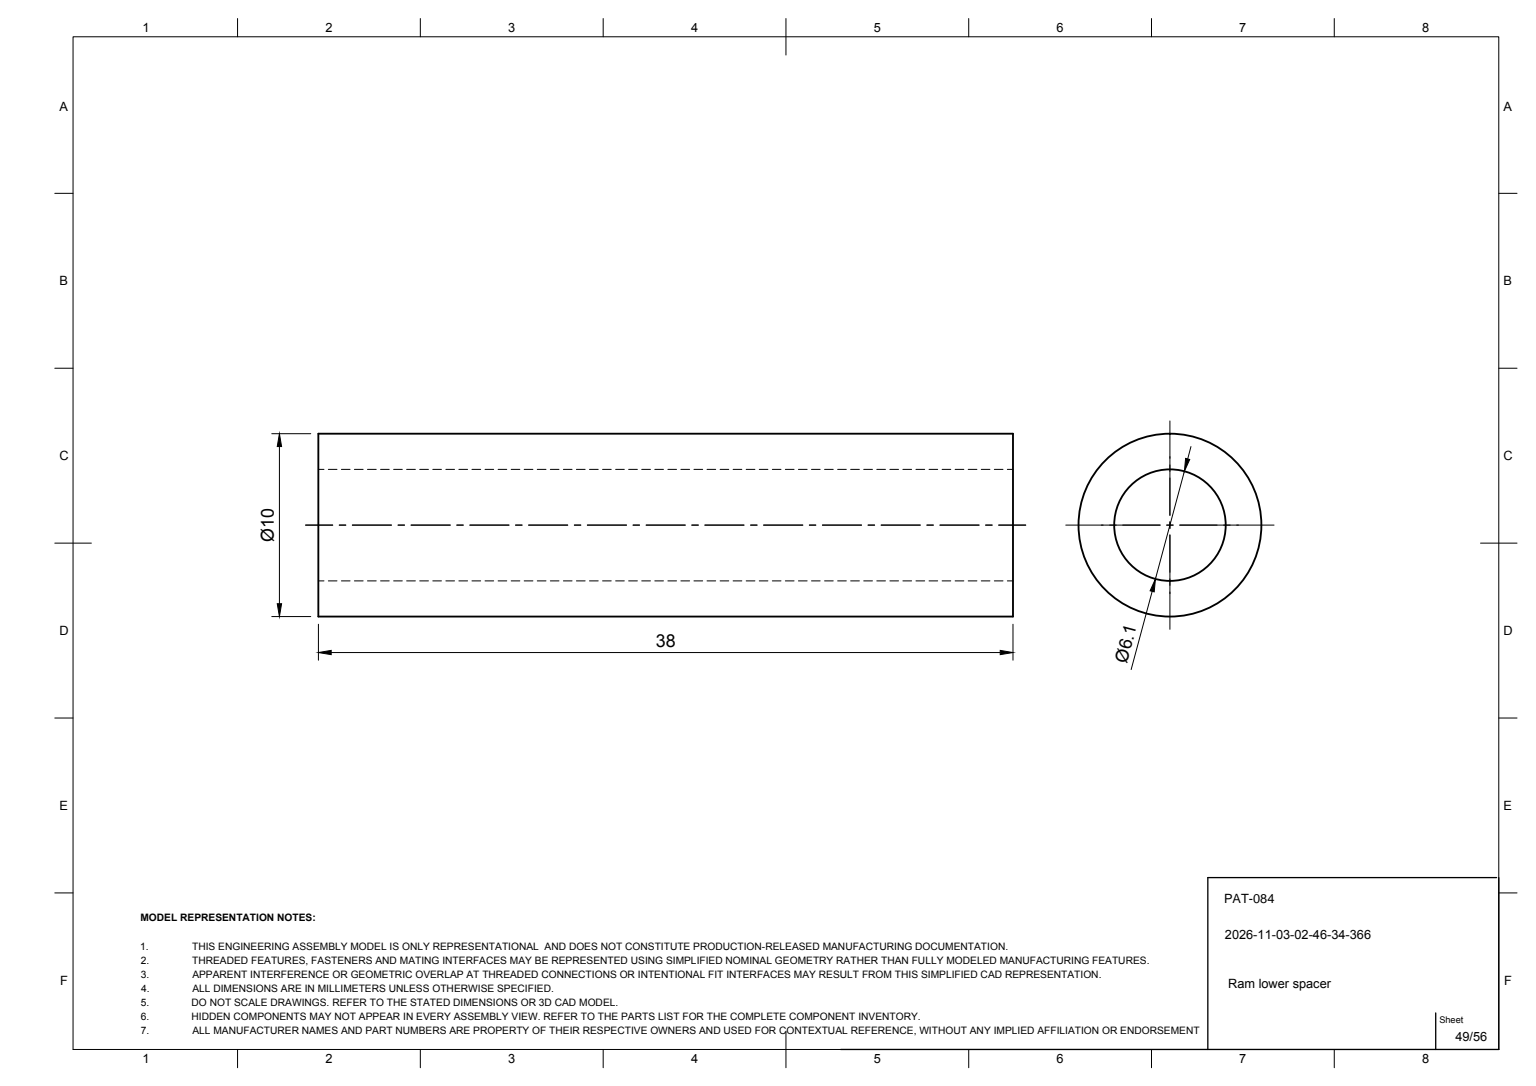
ISO-10303-21;
HEADER;
/* Generated by software containing ST-Developer
 * from STEP Tools, Inc. (www.steptools.com) 
 */

FILE_DESCRIPTION(
/* description */ ('Quick-return (Whitworth) mechanism'),
/* implementation_level */ '2;1');

FILE_NAME(
/* name */ 'Ram lower spacer.step',
/* time_stamp */ '2026-10-28T03:25:57-07:00',
/* author */ (''),
/* organization */ (''),
/* preprocessor_version */ 'ST-DEVELOPER v20.2',
/* originating_system */ 'Autodesk Translation Framework v15.17.0.0',
/* authorisation */ '');

FILE_SCHEMA (('AUTOMOTIVE_DESIGN { 1 0 10303 214 3 1 1 }'));
ENDSEC;

DATA;
#10=MECHANICAL_DESIGN_GEOMETRIC_PRESENTATION_REPRESENTATION('',(#534),#14878);
#438=SHAPE_REPRESENTATION_RELATIONSHIP('SRR','None',#15112,#482);
#482=ADVANCED_BREP_SHAPE_REPRESENTATION('',(#585),#14869);
#534=STYLED_ITEM('',(#15399),#585);
#585=MANIFOLD_SOLID_BREP('Body1',#7889);
#770=FACE_BOUND('',#2075,.T.);
#771=FACE_BOUND('',#2077,.T.);
#981=PLANE('',#9197);
#982=PLANE('',#9198);
#1427=FACE_OUTER_BOUND('',#2072,.T.);
#1428=FACE_OUTER_BOUND('',#2073,.T.);
#1429=FACE_OUTER_BOUND('',#2074,.T.);
#1430=FACE_OUTER_BOUND('',#2076,.T.);
#2072=EDGE_LOOP('',(#6814,#6815,#6816,#6817));
#2073=EDGE_LOOP('',(#6818,#6819,#6820,#6821));
#2074=EDGE_LOOP('',(#6822));
#2075=EDGE_LOOP('',(#6823));
#2076=EDGE_LOOP('',(#6824));
#2077=EDGE_LOOP('',(#6825));
#2537=LINE('',#14283,#3060);
#2538=LINE('',#14289,#3061);
#3060=VECTOR('',#11382,0.305);
#3061=VECTOR('',#11389,0.5);
#3589=CIRCLE('',#9192,0.305);
#3590=CIRCLE('',#9193,0.305);
#3591=CIRCLE('',#9195,0.5);
#3592=CIRCLE('',#9196,0.5);
#4158=VERTEX_POINT('',#14280);
#4159=VERTEX_POINT('',#14282);
#4160=VERTEX_POINT('',#14286);
#4161=VERTEX_POINT('',#14288);
#5064=EDGE_CURVE('',#4158,#4158,#3589,.T.);
#5065=EDGE_CURVE('',#4158,#4159,#2537,.T.);
#5066=EDGE_CURVE('',#4159,#4159,#3590,.T.);
#5067=EDGE_CURVE('',#4160,#4160,#3591,.T.);
#5068=EDGE_CURVE('',#4160,#4161,#2538,.T.);
#5069=EDGE_CURVE('',#4161,#4161,#3592,.T.);
#6814=ORIENTED_EDGE('',*,*,#5064,.F.);
#6815=ORIENTED_EDGE('',*,*,#5065,.T.);
#6816=ORIENTED_EDGE('',*,*,#5066,.T.);
#6817=ORIENTED_EDGE('',*,*,#5065,.F.);
#6818=ORIENTED_EDGE('',*,*,#5067,.F.);
#6819=ORIENTED_EDGE('',*,*,#5068,.T.);
#6820=ORIENTED_EDGE('',*,*,#5069,.T.);
#6821=ORIENTED_EDGE('',*,*,#5068,.F.);
#6822=ORIENTED_EDGE('',*,*,#5067,.T.);
#6823=ORIENTED_EDGE('',*,*,#5064,.T.);
#6824=ORIENTED_EDGE('',*,*,#5069,.F.);
#6825=ORIENTED_EDGE('',*,*,#5066,.F.);
#7364=CYLINDRICAL_SURFACE('',#9191,0.305);
#7365=CYLINDRICAL_SURFACE('',#9194,0.5);
#7758=ADVANCED_FACE('',(#1427),#7364,.F.);
#7759=ADVANCED_FACE('',(#1428),#7365,.T.);
#7760=ADVANCED_FACE('',(#1429,#770),#981,.T.);
#7761=ADVANCED_FACE('',(#1430,#771),#982,.F.);
#7889=CLOSED_SHELL('',(#7758,#7759,#7760,#7761));
#9190=AXIS2_PLACEMENT_3D('',#14278,#11376,#11377);
#9191=AXIS2_PLACEMENT_3D('',#14279,#11378,#11379);
#9192=AXIS2_PLACEMENT_3D('',#14281,#11380,#11381);
#9193=AXIS2_PLACEMENT_3D('',#14284,#11383,#11384);
#9194=AXIS2_PLACEMENT_3D('',#14285,#11385,#11386);
#9195=AXIS2_PLACEMENT_3D('',#14287,#11387,#11388);
#9196=AXIS2_PLACEMENT_3D('',#14290,#11390,#11391);
#9197=AXIS2_PLACEMENT_3D('',#14291,#11392,#11393);
#9198=AXIS2_PLACEMENT_3D('',#14292,#11394,#11395);
#11376=DIRECTION('axis',(0.,0.,1.));
#11377=DIRECTION('refdir',(1.,0.,0.));
#11378=DIRECTION('center_axis',(0.,0.,1.));
#11379=DIRECTION('ref_axis',(1.,0.,0.));
#11380=DIRECTION('center_axis',(0.,0.,-1.));
#11381=DIRECTION('ref_axis',(1.,0.,0.));
#11382=DIRECTION('',(0.,0.,-1.));
#11383=DIRECTION('center_axis',(0.,0.,-1.));
#11384=DIRECTION('ref_axis',(1.,0.,0.));
#11385=DIRECTION('center_axis',(0.,0.,1.));
#11386=DIRECTION('ref_axis',(1.,0.,0.));
#11387=DIRECTION('center_axis',(0.,0.,1.));
#11388=DIRECTION('ref_axis',(1.,0.,0.));
#11389=DIRECTION('',(0.,0.,-1.));
#11390=DIRECTION('center_axis',(0.,0.,1.));
#11391=DIRECTION('ref_axis',(1.,0.,0.));
#11392=DIRECTION('center_axis',(0.,0.,1.));
#11393=DIRECTION('ref_axis',(1.,0.,0.));
#11394=DIRECTION('center_axis',(0.,0.,1.));
#11395=DIRECTION('ref_axis',(1.,0.,0.));
#14278=CARTESIAN_POINT('',(0.,0.,0.));
#14279=CARTESIAN_POINT('Origin',(9.16515138991168,16.,4.6));
#14280=CARTESIAN_POINT('',(8.86015138991168,16.,8.4));
#14281=CARTESIAN_POINT('Origin',(9.16515138991168,16.,8.4));
#14282=CARTESIAN_POINT('',(8.86015138991168,16.,4.6));
#14283=CARTESIAN_POINT('',(8.86015138991168,16.,4.6));
#14284=CARTESIAN_POINT('Origin',(9.16515138991168,16.,4.6));
#14285=CARTESIAN_POINT('Origin',(9.16515138991168,16.,4.6));
#14286=CARTESIAN_POINT('',(8.66515138991168,16.,8.4));
#14287=CARTESIAN_POINT('Origin',(9.16515138991168,16.,8.4));
#14288=CARTESIAN_POINT('',(8.66515138991168,16.,4.6));
#14289=CARTESIAN_POINT('',(8.66515138991168,16.,4.6));
#14290=CARTESIAN_POINT('Origin',(9.16515138991168,16.,4.6));
#14291=CARTESIAN_POINT('Origin',(9.16515138991168,16.,8.4));
#14292=CARTESIAN_POINT('Origin',(9.16515138991168,16.,4.6));
#14815=UNCERTAINTY_MEASURE_WITH_UNIT(LENGTH_MEASURE(0.001),#14879,
'DISTANCE_ACCURACY_VALUE',
'Maximum model space distance between geometric entities at asserted c
onnectivities');
#14824=UNCERTAINTY_MEASURE_WITH_UNIT(LENGTH_MEASURE(0.001),#14879,
'DISTANCE_ACCURACY_VALUE',
'Maximum model space distance between geometric entities at asserted c
onnectivities');
#14869=(
GEOMETRIC_REPRESENTATION_CONTEXT(3)
GLOBAL_UNCERTAINTY_ASSIGNED_CONTEXT((#14815))
GLOBAL_UNIT_ASSIGNED_CONTEXT((#14879,#14881,#14882))
REPRESENTATION_CONTEXT('','3D')
);
#14878=(
GEOMETRIC_REPRESENTATION_CONTEXT(3)
GLOBAL_UNCERTAINTY_ASSIGNED_CONTEXT((#14824))
GLOBAL_UNIT_ASSIGNED_CONTEXT((#14879,#14881,#14882))
REPRESENTATION_CONTEXT('','3D')
);
#14879=(
LENGTH_UNIT()
NAMED_UNIT(*)
SI_UNIT(.CENTI.,.METRE.)
);
#14881=(
NAMED_UNIT(*)
PLANE_ANGLE_UNIT()
SI_UNIT($,.RADIAN.)
);
#14882=(
NAMED_UNIT(*)
SI_UNIT($,.STERADIAN.)
SOLID_ANGLE_UNIT()
);
#14927=SHAPE_DEFINITION_REPRESENTATION(#14989,#15112);
#14989=PRODUCT_DEFINITION_SHAPE('',$,#15166);
#15112=SHAPE_REPRESENTATION('',(#9190),#14869);
#15121=PRODUCT_DEFINITION_CONTEXT('part definition',#15282,'design');
#15166=PRODUCT_DEFINITION('Ram lower spacer','Ram lower spacer',#15219,
#15121);
#15219=PRODUCT_DEFINITION_FORMATION('',$,#15328);
#15282=APPLICATION_CONTEXT(
'Core Data for Automotive Mechanical Design Process');
#15283=PRODUCT_CONTEXT('part definition',#15282,'mechanical');
#15328=PRODUCT('Ram lower spacer','Ram lower spacer','Ram lower spacer',
(#15283));
#15393=COLOUR_RGB('Sky Blue',0.24,0.69,0.87);
#15394=FILL_AREA_STYLE_COLOUR('',#15393);
#15395=FILL_AREA_STYLE('',(#15394));
#15396=SURFACE_STYLE_FILL_AREA(#15395);
#15397=SURFACE_SIDE_STYLE('',(#15396));
#15398=SURFACE_STYLE_USAGE(.BOTH.,#15397);
#15399=PRESENTATION_STYLE_ASSIGNMENT((#15398));
ENDSEC;
END-ISO-10303-21;
